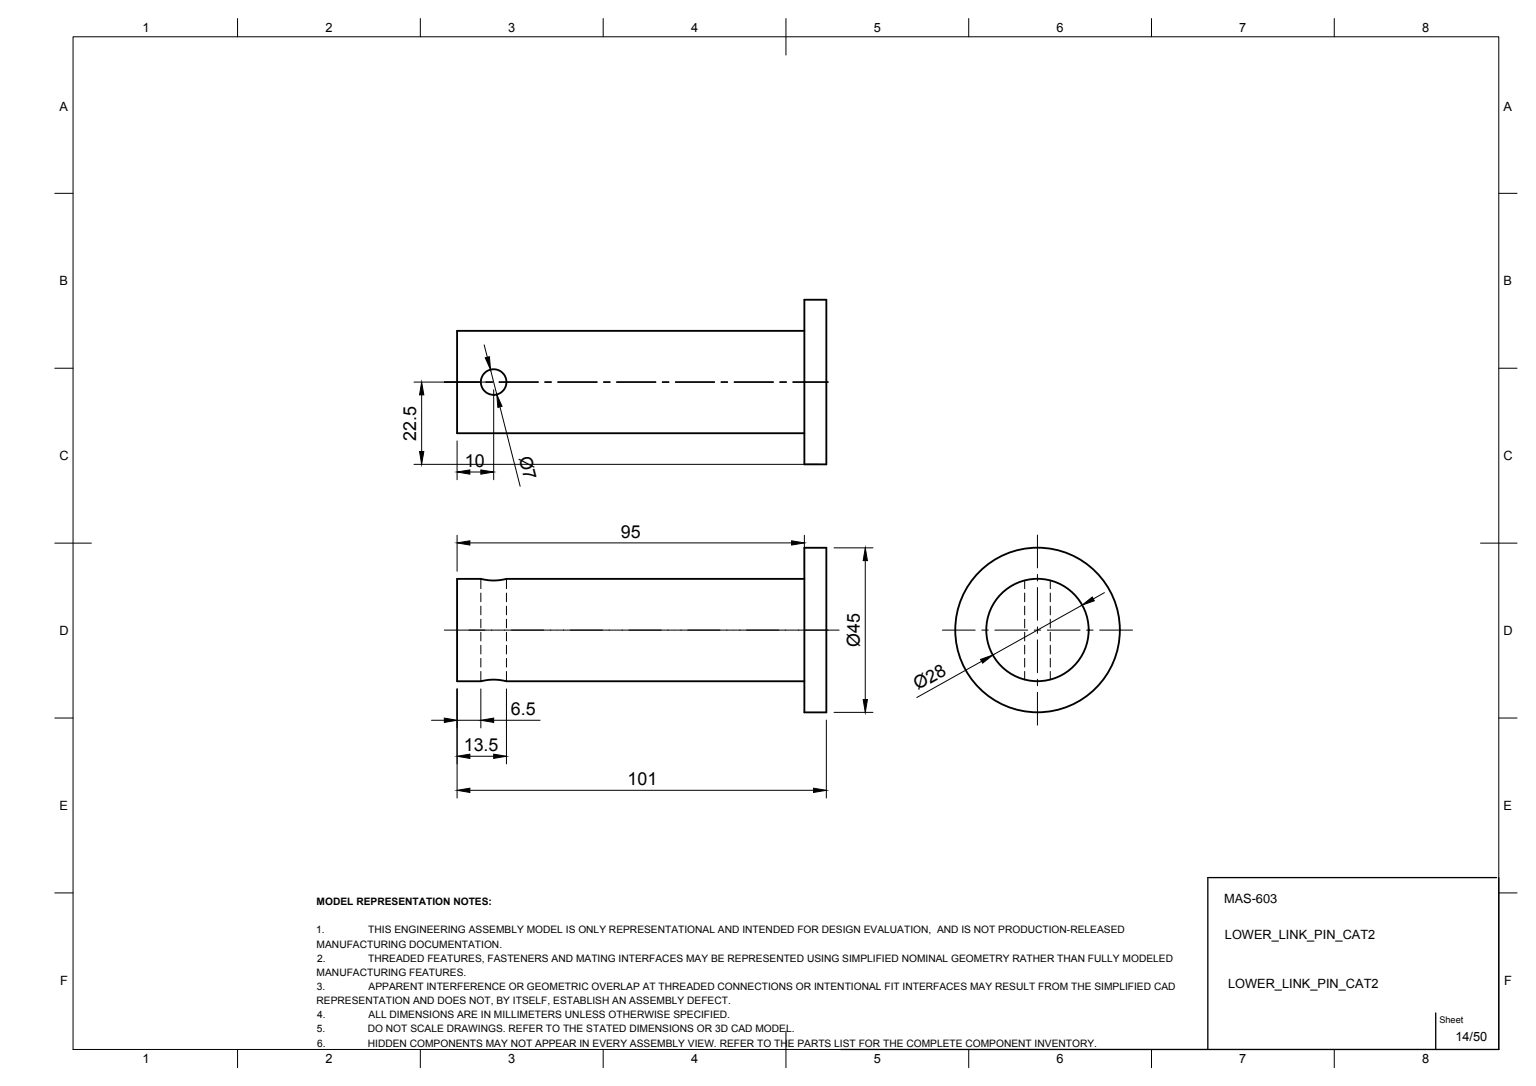
ISO-10303-21;
HEADER;
FILE_DESCRIPTION((''),'2;1');
FILE_NAME('LOWER_LINK_PIN_CAT2.step','2026-10-01T22:06:14-07:00',(''),(''),'','','');
FILE_SCHEMA (('AUTOMOTIVE_DESIGN { 1 0 10303 214 3 1 1 }'));
ENDSEC;
DATA;
#10=MECHANICAL_DESIGN_GEOMETRIC_PRESENTATION_REPRESENTATION('',(#988),#50440);
#11=B_SPLINE_CURVE_WITH_KNOTS('',3,(#44873,#44874,#44875,#44876,#44877,
#44878,#44879,#44880,#44881,#44882,#44883,#44884,#44885,#44886,#44887,#44888,
#44889,#44890),.UNSPECIFIED.,.F.,.F.,(4,2,2,2,2,2,2,2,4),(0.,0.13245688121231,
0.264913762424621,0.39735212380502,0.529790485185418,0.662228846565817,
0.794667207946216,0.927124089158526,1.05958097037084),.UNSPECIFIED.) ;
#12=B_SPLINE_CURVE_WITH_KNOTS('',3,(#44891,#44892,#44893,#44894,#44895,
#44896,#44897,#44898,#44899,#44900,#44901,#44902,#44903,#44904,#44905,#44906,
#44907,#44908),.UNSPECIFIED.,.F.,.F.,(4,2,2,2,2,2,2,2,4),(1.05958097037084,
1.19203785158315,1.32449473279546,1.45693309417586,1.58937145555626,1.72180981693665,
1.85424817831705,1.98670505952936,2.11916194074167),.UNSPECIFIED.) ;
#13=B_SPLINE_CURVE_WITH_KNOTS('',3,(#44912,#44913,#44914,#44915,#44916,
#44917,#44918,#44919,#44920,#44921,#44922,#44923,#44924,#44925,#44926,#44927,
#44928,#44929),.UNSPECIFIED.,.F.,.F.,(4,2,2,2,2,2,2,2,4),(0.,0.13245688121231,
0.264913762424621,0.39735212380502,0.529790485185418,0.662228846565817,
0.794667207946216,0.927124089158526,1.05958097037084),.UNSPECIFIED.) ;
#14=B_SPLINE_CURVE_WITH_KNOTS('',3,(#44930,#44931,#44932,#44933,#44934,
#44935,#44936,#44937,#44938,#44939,#44940,#44941,#44942,#44943,#44944,#44945,
#44946,#44947),.UNSPECIFIED.,.F.,.F.,(4,2,2,2,2,2,2,2,4),(1.05958097037084,
1.19203785158315,1.32449473279546,1.45693309417586,1.58937145555626,1.72180981693665,
1.85424817831705,1.98670505952936,2.11916194074167),.UNSPECIFIED.) ;
#898=SHAPE_REPRESENTATION_RELATIONSHIP('SRR','None',#50629,#943) ;
#943=ADVANCED_BREP_SHAPE_REPRESENTATION('',(#1043),#50398) ;
#988=STYLED_ITEM('',(#50883),#1043) ;
#1043=MANIFOLD_SOLID_BREP('LOWER_LINK_PIN_CAT2',#28655) ;
#1270=FACE_BOUND('',#4727,.T.) ;
#1271=FACE_BOUND('',#4731,.T.) ;
#1272=FACE_BOUND('',#4732,.T.) ;
#1926=PLANE('',#30255) ;
#1927=PLANE('',#30260) ;
#1928=PLANE('',#30263) ;
#3013=FACE_OUTER_BOUND('',#4725,.T.) ;
#3014=FACE_OUTER_BOUND('',#4726,.T.) ;
#3015=FACE_OUTER_BOUND('',#4728,.T.) ;
#3016=FACE_OUTER_BOUND('',#4729,.T.) ;
#3017=FACE_OUTER_BOUND('',#4730,.T.) ;
#3018=FACE_OUTER_BOUND('',#4733,.T.) ;
#4725=EDGE_LOOP('',(#22111,#22112,#22113,#22114,#22115,#22116)) ;
#4726=EDGE_LOOP('',(#22117)) ;
#4727=EDGE_LOOP('',(#22118)) ;
#4728=EDGE_LOOP('',(#22119,#22120,#22121,#22122)) ;
#4729=EDGE_LOOP('',(#22123)) ;
#4730=EDGE_LOOP('',(#22124,#22125,#22126,#22127)) ;
#4731=EDGE_LOOP('',(#22128,#22129)) ;
#4732=EDGE_LOOP('',(#22130,#22131)) ;
#4733=EDGE_LOOP('',(#22132)) ;
#7135=LINE('',#44910,#9607) ;
#7136=LINE('',#44955,#9608) ;
#7137=LINE('',#44961,#9609) ;
#9607=VECTOR('',#35870,0.35) ;
#9608=VECTOR('',#35879,2.25) ;
#9609=VECTOR('',#35888,1.4) ;
#10998=CIRCLE('',#30256,2.25) ;
#10999=CIRCLE('',#30257,1.4) ;
#11000=CIRCLE('',#30259,2.25) ;
#11001=CIRCLE('',#30262,1.4) ;
#13020=VERTEX_POINT('',#44871) ;
#13021=VERTEX_POINT('',#44872) ;
#13022=VERTEX_POINT('',#44909) ;
#13023=VERTEX_POINT('',#44911) ;
#13024=VERTEX_POINT('',#44949) ;
#13025=VERTEX_POINT('',#44951) ;
#13026=VERTEX_POINT('',#44954) ;
#13027=VERTEX_POINT('',#44959) ;
#16321=EDGE_CURVE('',#13020,#13021,#11,.T.) ;
#16322=EDGE_CURVE('',#13021,#13020,#12,.T.) ;
#16323=EDGE_CURVE('',#13021,#13022,#7135,.T.) ;
#16324=EDGE_CURVE('',#13023,#13022,#13,.T.) ;
#16325=EDGE_CURVE('',#13022,#13023,#14,.T.) ;
#16326=EDGE_CURVE('',#13024,#13024,#10998,.T.) ;
#16327=EDGE_CURVE('',#13025,#13025,#10999,.T.) ;
#16328=EDGE_CURVE('',#13024,#13026,#7136,.T.) ;
#16329=EDGE_CURVE('',#13026,#13026,#11000,.T.) ;
#16330=EDGE_CURVE('',#13027,#13027,#11001,.T.) ;
#16331=EDGE_CURVE('',#13027,#13025,#7137,.T.) ;
#22111=ORIENTED_EDGE('',*,*,#16321,.F.) ;
#22112=ORIENTED_EDGE('',*,*,#16322,.F.) ;
#22113=ORIENTED_EDGE('',*,*,#16323,.T.) ;
#22114=ORIENTED_EDGE('',*,*,#16324,.F.) ;
#22115=ORIENTED_EDGE('',*,*,#16325,.F.) ;
#22116=ORIENTED_EDGE('',*,*,#16323,.F.) ;
#22117=ORIENTED_EDGE('',*,*,#16326,.T.) ;
#22118=ORIENTED_EDGE('',*,*,#16327,.T.) ;
#22119=ORIENTED_EDGE('',*,*,#16326,.F.) ;
#22120=ORIENTED_EDGE('',*,*,#16328,.T.) ;
#22121=ORIENTED_EDGE('',*,*,#16329,.F.) ;
#22122=ORIENTED_EDGE('',*,*,#16328,.F.) ;
#22123=ORIENTED_EDGE('',*,*,#16329,.T.) ;
#22124=ORIENTED_EDGE('',*,*,#16330,.F.) ;
#22125=ORIENTED_EDGE('',*,*,#16331,.T.) ;
#22126=ORIENTED_EDGE('',*,*,#16327,.F.) ;
#22127=ORIENTED_EDGE('',*,*,#16331,.F.) ;
#22128=ORIENTED_EDGE('',*,*,#16324,.T.) ;
#22129=ORIENTED_EDGE('',*,*,#16325,.T.) ;
#22130=ORIENTED_EDGE('',*,*,#16321,.T.) ;
#22131=ORIENTED_EDGE('',*,*,#16322,.T.) ;
#22132=ORIENTED_EDGE('',*,*,#16330,.T.) ;
#26776=CYLINDRICAL_SURFACE('',#30254,0.35) ;
#26777=CYLINDRICAL_SURFACE('',#30258,2.25) ;
#26778=CYLINDRICAL_SURFACE('',#30261,1.4) ;
#27748=ADVANCED_FACE('',(#3013),#26776,.F.) ;
#27749=ADVANCED_FACE('',(#3014,#1270),#1926,.T.) ;
#27750=ADVANCED_FACE('',(#3015),#26777,.T.) ;
#27751=ADVANCED_FACE('',(#3016),#1927,.T.) ;
#27752=ADVANCED_FACE('',(#3017,#1271,#1272),#26778,.T.) ;
#27753=ADVANCED_FACE('',(#3018),#1928,.T.) ;
#28655=CLOSED_SHELL('',(#27748,#27749,#27750,#27751,#27752,#27753)) ;
#30253=AXIS2_PLACEMENT_3D('',#44869,#35866,#35867) ;
#30254=AXIS2_PLACEMENT_3D('',#44870,#35868,#35869) ;
#30255=AXIS2_PLACEMENT_3D('',#44948,#35871,#35872) ;
#30256=AXIS2_PLACEMENT_3D('',#44950,#35873,#35874) ;
#30257=AXIS2_PLACEMENT_3D('',#44952,#35875,#35876) ;
#30258=AXIS2_PLACEMENT_3D('',#44953,#35877,#35878) ;
#30259=AXIS2_PLACEMENT_3D('',#44956,#35880,#35881) ;
#30260=AXIS2_PLACEMENT_3D('',#44957,#35882,#35883) ;
#30261=AXIS2_PLACEMENT_3D('',#44958,#35884,#35885) ;
#30262=AXIS2_PLACEMENT_3D('',#44960,#35886,#35887) ;
#30263=AXIS2_PLACEMENT_3D('',#44962,#35889,#35890) ;
#35866=DIRECTION('axis',(0.,0.,1.)) ;
#35867=DIRECTION('refdir',(1.,0.,0.)) ;
#35868=DIRECTION('center_axis',(0.,0.,1.)) ;
#35869=DIRECTION('ref_axis',(1.,0.,0.)) ;
#35870=DIRECTION('',(0.,0.,1.)) ;
#35871=DIRECTION('center_axis',(0.,1.,0.)) ;
#35872=DIRECTION('ref_axis',(1.,0.,0.)) ;
#35873=DIRECTION('center_axis',(0.,1.,0.)) ;
#35874=DIRECTION('ref_axis',(1.,0.,0.)) ;
#35875=DIRECTION('center_axis',(0.,-1.,0.)) ;
#35876=DIRECTION('ref_axis',(1.,0.,0.)) ;
#35877=DIRECTION('center_axis',(0.,1.,0.)) ;
#35878=DIRECTION('ref_axis',(1.,0.,0.)) ;
#35879=DIRECTION('',(0.,-1.,0.)) ;
#35880=DIRECTION('center_axis',(0.,-1.,0.)) ;
#35881=DIRECTION('ref_axis',(1.,0.,0.)) ;
#35882=DIRECTION('center_axis',(0.,-1.,0.)) ;
#35883=DIRECTION('ref_axis',(-1.,0.,0.)) ;
#35884=DIRECTION('center_axis',(0.,1.,0.)) ;
#35885=DIRECTION('ref_axis',(1.,0.,0.)) ;
#35886=DIRECTION('center_axis',(0.,1.,0.)) ;
#35887=DIRECTION('ref_axis',(1.,0.,0.)) ;
#35888=DIRECTION('',(0.,-1.,0.)) ;
#35889=DIRECTION('center_axis',(0.,1.,0.)) ;
#35890=DIRECTION('ref_axis',(1.,0.,0.)) ;
#44869=CARTESIAN_POINT('',(0.,0.,0.)) ;
#44870=CARTESIAN_POINT('Origin',(0.,8.5,0.)) ;
#44871=CARTESIAN_POINT('',(0.35,8.5,-1.3555441711726)) ;
#44872=CARTESIAN_POINT('',(-0.35,8.5,-1.3555441711726)) ;
#44873=CARTESIAN_POINT('Ctrl Pts',(0.35,8.5,-1.3555441711726)) ;
#44874=CARTESIAN_POINT('Ctrl Pts',(0.35,8.54415229373744,-1.3555441711726)) ;
#44875=CARTESIAN_POINT('Ctrl Pts',(0.341137668931484,8.59111259780368,-1.3579260221299)) ;
#44876=CARTESIAN_POINT('Ctrl Pts',(0.305362394790648,8.67728573976065,-1.36641567222626)) ;
#44877=CARTESIAN_POINT('Ctrl Pts',(0.278458987739036,8.71651575909155,-1.37238871180719)) ;
#44878=CARTESIAN_POINT('Ctrl Pts',(0.216520089475035,8.77845465735555,-1.38351326633711)) ;
#44879=CARTESIAN_POINT('Ctrl Pts',(0.177288266610716,8.80536144075754,-1.38940376323118)) ;
#44880=CARTESIAN_POINT('Ctrl Pts',(0.0911087295357738,8.84113917986052,
-1.39770281034285)) ;
#44881=CARTESIAN_POINT('Ctrl Pts',(0.0441461204601329,8.85,-1.4)) ;
#44882=CARTESIAN_POINT('Ctrl Pts',(-0.0441461204601329,8.85,-1.4)) ;
#44883=CARTESIAN_POINT('Ctrl Pts',(-0.0911087295357738,8.84113917986052,
-1.39770281034285)) ;
#44884=CARTESIAN_POINT('Ctrl Pts',(-0.177288266610716,8.80536144075754,
-1.38940376323118)) ;
#44885=CARTESIAN_POINT('Ctrl Pts',(-0.216520089475035,8.77845465735555,
-1.38351326633711)) ;
#44886=CARTESIAN_POINT('Ctrl Pts',(-0.278458987739036,8.71651575909155,
-1.37238871180719)) ;
#44887=CARTESIAN_POINT('Ctrl Pts',(-0.305362394790648,8.67728573976065,
-1.36641567222626)) ;
#44888=CARTESIAN_POINT('Ctrl Pts',(-0.341137668931484,8.59111259780368,
-1.3579260221299)) ;
#44889=CARTESIAN_POINT('Ctrl Pts',(-0.35,8.54415229373744,-1.3555441711726)) ;
#44890=CARTESIAN_POINT('Ctrl Pts',(-0.35,8.5,-1.3555441711726)) ;
#44891=CARTESIAN_POINT('Ctrl Pts',(-0.35,8.5,-1.3555441711726)) ;
#44892=CARTESIAN_POINT('Ctrl Pts',(-0.35,8.45584770626256,-1.3555441711726)) ;
#44893=CARTESIAN_POINT('Ctrl Pts',(-0.341137668931484,8.40888740219632,
-1.3579260221299)) ;
#44894=CARTESIAN_POINT('Ctrl Pts',(-0.305362394790648,8.32271426023935,
-1.36641567222626)) ;
#44895=CARTESIAN_POINT('Ctrl Pts',(-0.278458987739036,8.28348424090845,
-1.37238871180719)) ;
#44896=CARTESIAN_POINT('Ctrl Pts',(-0.216520089475035,8.22154534264445,
-1.38351326633711)) ;
#44897=CARTESIAN_POINT('Ctrl Pts',(-0.177288266610716,8.19463855924246,
-1.38940376323118)) ;
#44898=CARTESIAN_POINT('Ctrl Pts',(-0.0911087295357738,8.15886082013948,
-1.39770281034285)) ;
#44899=CARTESIAN_POINT('Ctrl Pts',(-0.044146120460133,8.15,-1.4)) ;
#44900=CARTESIAN_POINT('Ctrl Pts',(0.0441461204601329,8.15,-1.4)) ;
#44901=CARTESIAN_POINT('Ctrl Pts',(0.0911087295357739,8.15886082013948,
-1.39770281034285)) ;
#44902=CARTESIAN_POINT('Ctrl Pts',(0.177288266610716,8.19463855924246,-1.38940376323118)) ;
#44903=CARTESIAN_POINT('Ctrl Pts',(0.216520089475035,8.22154534264445,-1.38351326633711)) ;
#44904=CARTESIAN_POINT('Ctrl Pts',(0.278458987739037,8.28348424090845,-1.37238871180719)) ;
#44905=CARTESIAN_POINT('Ctrl Pts',(0.305362394790648,8.32271426023935,-1.36641567222626)) ;
#44906=CARTESIAN_POINT('Ctrl Pts',(0.341137668931484,8.40888740219632,-1.3579260221299)) ;
#44907=CARTESIAN_POINT('Ctrl Pts',(0.35,8.45584770626257,-1.3555441711726)) ;
#44908=CARTESIAN_POINT('Ctrl Pts',(0.35,8.5,-1.3555441711726)) ;
#44909=CARTESIAN_POINT('',(-0.35,8.5,1.3555441711726)) ;
#44910=CARTESIAN_POINT('',(-0.35,8.5,0.)) ;
#44911=CARTESIAN_POINT('',(0.35,8.5,1.3555441711726)) ;
#44912=CARTESIAN_POINT('Ctrl Pts',(0.35,8.5,1.3555441711726)) ;
#44913=CARTESIAN_POINT('Ctrl Pts',(0.35,8.45584770626256,1.3555441711726)) ;
#44914=CARTESIAN_POINT('Ctrl Pts',(0.341137668931484,8.40888740219632,1.3579260221299)) ;
#44915=CARTESIAN_POINT('Ctrl Pts',(0.305362394790648,8.32271426023935,1.36641567222626)) ;
#44916=CARTESIAN_POINT('Ctrl Pts',(0.278458987739037,8.28348424090845,1.37238871180719)) ;
#44917=CARTESIAN_POINT('Ctrl Pts',(0.216520089475035,8.22154534264445,1.38351326633711)) ;
#44918=CARTESIAN_POINT('Ctrl Pts',(0.177288266610716,8.19463855924246,1.38940376323118)) ;
#44919=CARTESIAN_POINT('Ctrl Pts',(0.0911087295357738,8.15886082013948,
1.39770281034285)) ;
#44920=CARTESIAN_POINT('Ctrl Pts',(0.0441461204601329,8.15,1.4)) ;
#44921=CARTESIAN_POINT('Ctrl Pts',(-0.044146120460133,8.15,1.4)) ;
#44922=CARTESIAN_POINT('Ctrl Pts',(-0.0911087295357739,8.15886082013948,
1.39770281034285)) ;
#44923=CARTESIAN_POINT('Ctrl Pts',(-0.177288266610716,8.19463855924246,
1.38940376323118)) ;
#44924=CARTESIAN_POINT('Ctrl Pts',(-0.216520089475035,8.22154534264445,
1.38351326633711)) ;
#44925=CARTESIAN_POINT('Ctrl Pts',(-0.278458987739036,8.28348424090845,
1.37238871180719)) ;
#44926=CARTESIAN_POINT('Ctrl Pts',(-0.305362394790648,8.32271426023935,
1.36641567222626)) ;
#44927=CARTESIAN_POINT('Ctrl Pts',(-0.341137668931484,8.40888740219632,
1.3579260221299)) ;
#44928=CARTESIAN_POINT('Ctrl Pts',(-0.35,8.45584770626256,1.3555441711726)) ;
#44929=CARTESIAN_POINT('Ctrl Pts',(-0.35,8.5,1.3555441711726)) ;
#44930=CARTESIAN_POINT('Ctrl Pts',(-0.35,8.5,1.3555441711726)) ;
#44931=CARTESIAN_POINT('Ctrl Pts',(-0.35,8.54415229373744,1.3555441711726)) ;
#44932=CARTESIAN_POINT('Ctrl Pts',(-0.341137668931484,8.59111259780368,
1.3579260221299)) ;
#44933=CARTESIAN_POINT('Ctrl Pts',(-0.305362394790648,8.67728573976065,
1.36641567222626)) ;
#44934=CARTESIAN_POINT('Ctrl Pts',(-0.278458987739036,8.71651575909155,
1.37238871180719)) ;
#44935=CARTESIAN_POINT('Ctrl Pts',(-0.216520089475035,8.77845465735555,
1.38351326633711)) ;
#44936=CARTESIAN_POINT('Ctrl Pts',(-0.177288266610716,8.80536144075754,
1.38940376323118)) ;
#44937=CARTESIAN_POINT('Ctrl Pts',(-0.0911087295357738,8.84113917986052,
1.39770281034285)) ;
#44938=CARTESIAN_POINT('Ctrl Pts',(-0.0441461204601329,8.85,1.4)) ;
#44939=CARTESIAN_POINT('Ctrl Pts',(0.0441461204601329,8.85,1.4)) ;
#44940=CARTESIAN_POINT('Ctrl Pts',(0.0911087295357738,8.84113917986052,
1.39770281034285)) ;
#44941=CARTESIAN_POINT('Ctrl Pts',(0.177288266610716,8.80536144075754,1.38940376323118)) ;
#44942=CARTESIAN_POINT('Ctrl Pts',(0.216520089475035,8.77845465735555,1.38351326633711)) ;
#44943=CARTESIAN_POINT('Ctrl Pts',(0.278458987739036,8.71651575909155,1.37238871180719)) ;
#44944=CARTESIAN_POINT('Ctrl Pts',(0.305362394790648,8.67728573976065,1.36641567222626)) ;
#44945=CARTESIAN_POINT('Ctrl Pts',(0.341137668931484,8.59111259780368,1.3579260221299)) ;
#44946=CARTESIAN_POINT('Ctrl Pts',(0.35,8.54415229373743,1.3555441711726)) ;
#44947=CARTESIAN_POINT('Ctrl Pts',(0.35,8.5,1.3555441711726)) ;
#44948=CARTESIAN_POINT('Origin',(0.,0.,0.)) ;
#44949=CARTESIAN_POINT('',(-2.25,0.,2.75545529808154E-16)) ;
#44950=CARTESIAN_POINT('Origin',(0.,0.,0.)) ;
#44951=CARTESIAN_POINT('',(-1.4,0.,1.71450551880629E-16)) ;
#44952=CARTESIAN_POINT('Origin',(0.,0.,0.)) ;
#44953=CARTESIAN_POINT('Origin',(0.,-0.3,0.)) ;
#44954=CARTESIAN_POINT('',(-2.25,-0.6,2.75545529808154E-16)) ;
#44955=CARTESIAN_POINT('',(-2.25,-0.3,2.75545529808154E-16)) ;
#44956=CARTESIAN_POINT('Origin',(0.,-0.6,0.)) ;
#44957=CARTESIAN_POINT('Origin',(0.,-0.6,0.)) ;
#44958=CARTESIAN_POINT('Origin',(0.,4.75,0.)) ;
#44959=CARTESIAN_POINT('',(-1.4,9.5,1.71450551880629E-16)) ;
#44960=CARTESIAN_POINT('Origin',(0.,9.5,0.)) ;
#44961=CARTESIAN_POINT('',(-1.4,4.75,1.71450551880629E-16)) ;
#44962=CARTESIAN_POINT('Origin',(0.,9.5,0.)) ;
#50345=UNCERTAINTY_MEASURE_WITH_UNIT(LENGTH_MEASURE(0.001),#50441,
'DISTANCE_ACCURACY_VALUE',
'Maximum model space distance between geometric entities at asserted c
onnectivities') ;
#50387=UNCERTAINTY_MEASURE_WITH_UNIT(LENGTH_MEASURE(0.001),#50441,
'DISTANCE_ACCURACY_VALUE',
'Maximum model space distance between geometric entities at asserted c
onnectivities') ;
#50398=(
GEOMETRIC_REPRESENTATION_CONTEXT(3)
GLOBAL_UNCERTAINTY_ASSIGNED_CONTEXT((#50345))
GLOBAL_UNIT_ASSIGNED_CONTEXT((#50441,#50443,#50444))
REPRESENTATION_CONTEXT('','3D')
) ;
#50440=(
GEOMETRIC_REPRESENTATION_CONTEXT(3)
GLOBAL_UNCERTAINTY_ASSIGNED_CONTEXT((#50387))
GLOBAL_UNIT_ASSIGNED_CONTEXT((#50441,#50443,#50444))
REPRESENTATION_CONTEXT('','3D')
) ;
#50441=(
LENGTH_UNIT()
NAMED_UNIT(*)
SI_UNIT(.CENTI.,.METRE.)
) ;
#50443=(
NAMED_UNIT(*)
PLANE_ANGLE_UNIT()
SI_UNIT($,.RADIAN.)
) ;
#50444=(
NAMED_UNIT(*)
SI_UNIT($,.STERADIAN.)
SOLID_ANGLE_UNIT()
) ;
#50455=SHAPE_DEFINITION_REPRESENTATION(#50513,#50629) ;
#50513=PRODUCT_DEFINITION_SHAPE('',$,#50682) ;
#50629=SHAPE_REPRESENTATION('',(#30253),#50398) ;
#50671=PRODUCT_DEFINITION_CONTEXT('part definition',#50829,'design') ;
#50682=PRODUCT_DEFINITION('LOWER_LINK_PIN_CAT2',
'LOWER_LINK_PIN_CAT2',#50734,#50671) ;
#50734=PRODUCT_DEFINITION_FORMATION('',$,#50841) ;
#50829=APPLICATION_CONTEXT(
'Core Data for Automotive Mechanical Design Process') ;
#50830=PRODUCT_CONTEXT('part definition',#50829,'mechanical') ;
#50841=PRODUCT('LOWER_LINK_PIN_CAT2','LOWER_LINK_PIN_CAT2',$,(#50830)) ;
#50883=PRESENTATION_STYLE_ASSIGNMENT((#50890)) ;
#50890=SURFACE_STYLE_USAGE(.BOTH.,#50897) ;
#50897=SURFACE_SIDE_STYLE('',(#50904)) ;
#50904=SURFACE_STYLE_FILL_AREA(#50911) ;
#50911=FILL_AREA_STYLE('Steel - Satin',(#50918)) ;
#50918=FILL_AREA_STYLE_COLOUR('Steel - Satin',#50925) ;
#50925=COLOUR_RGB('Steel - Satin', 0.31764706, 0.68627451, 0.89019608) ;
ENDSEC;
END-ISO-10303-21;
